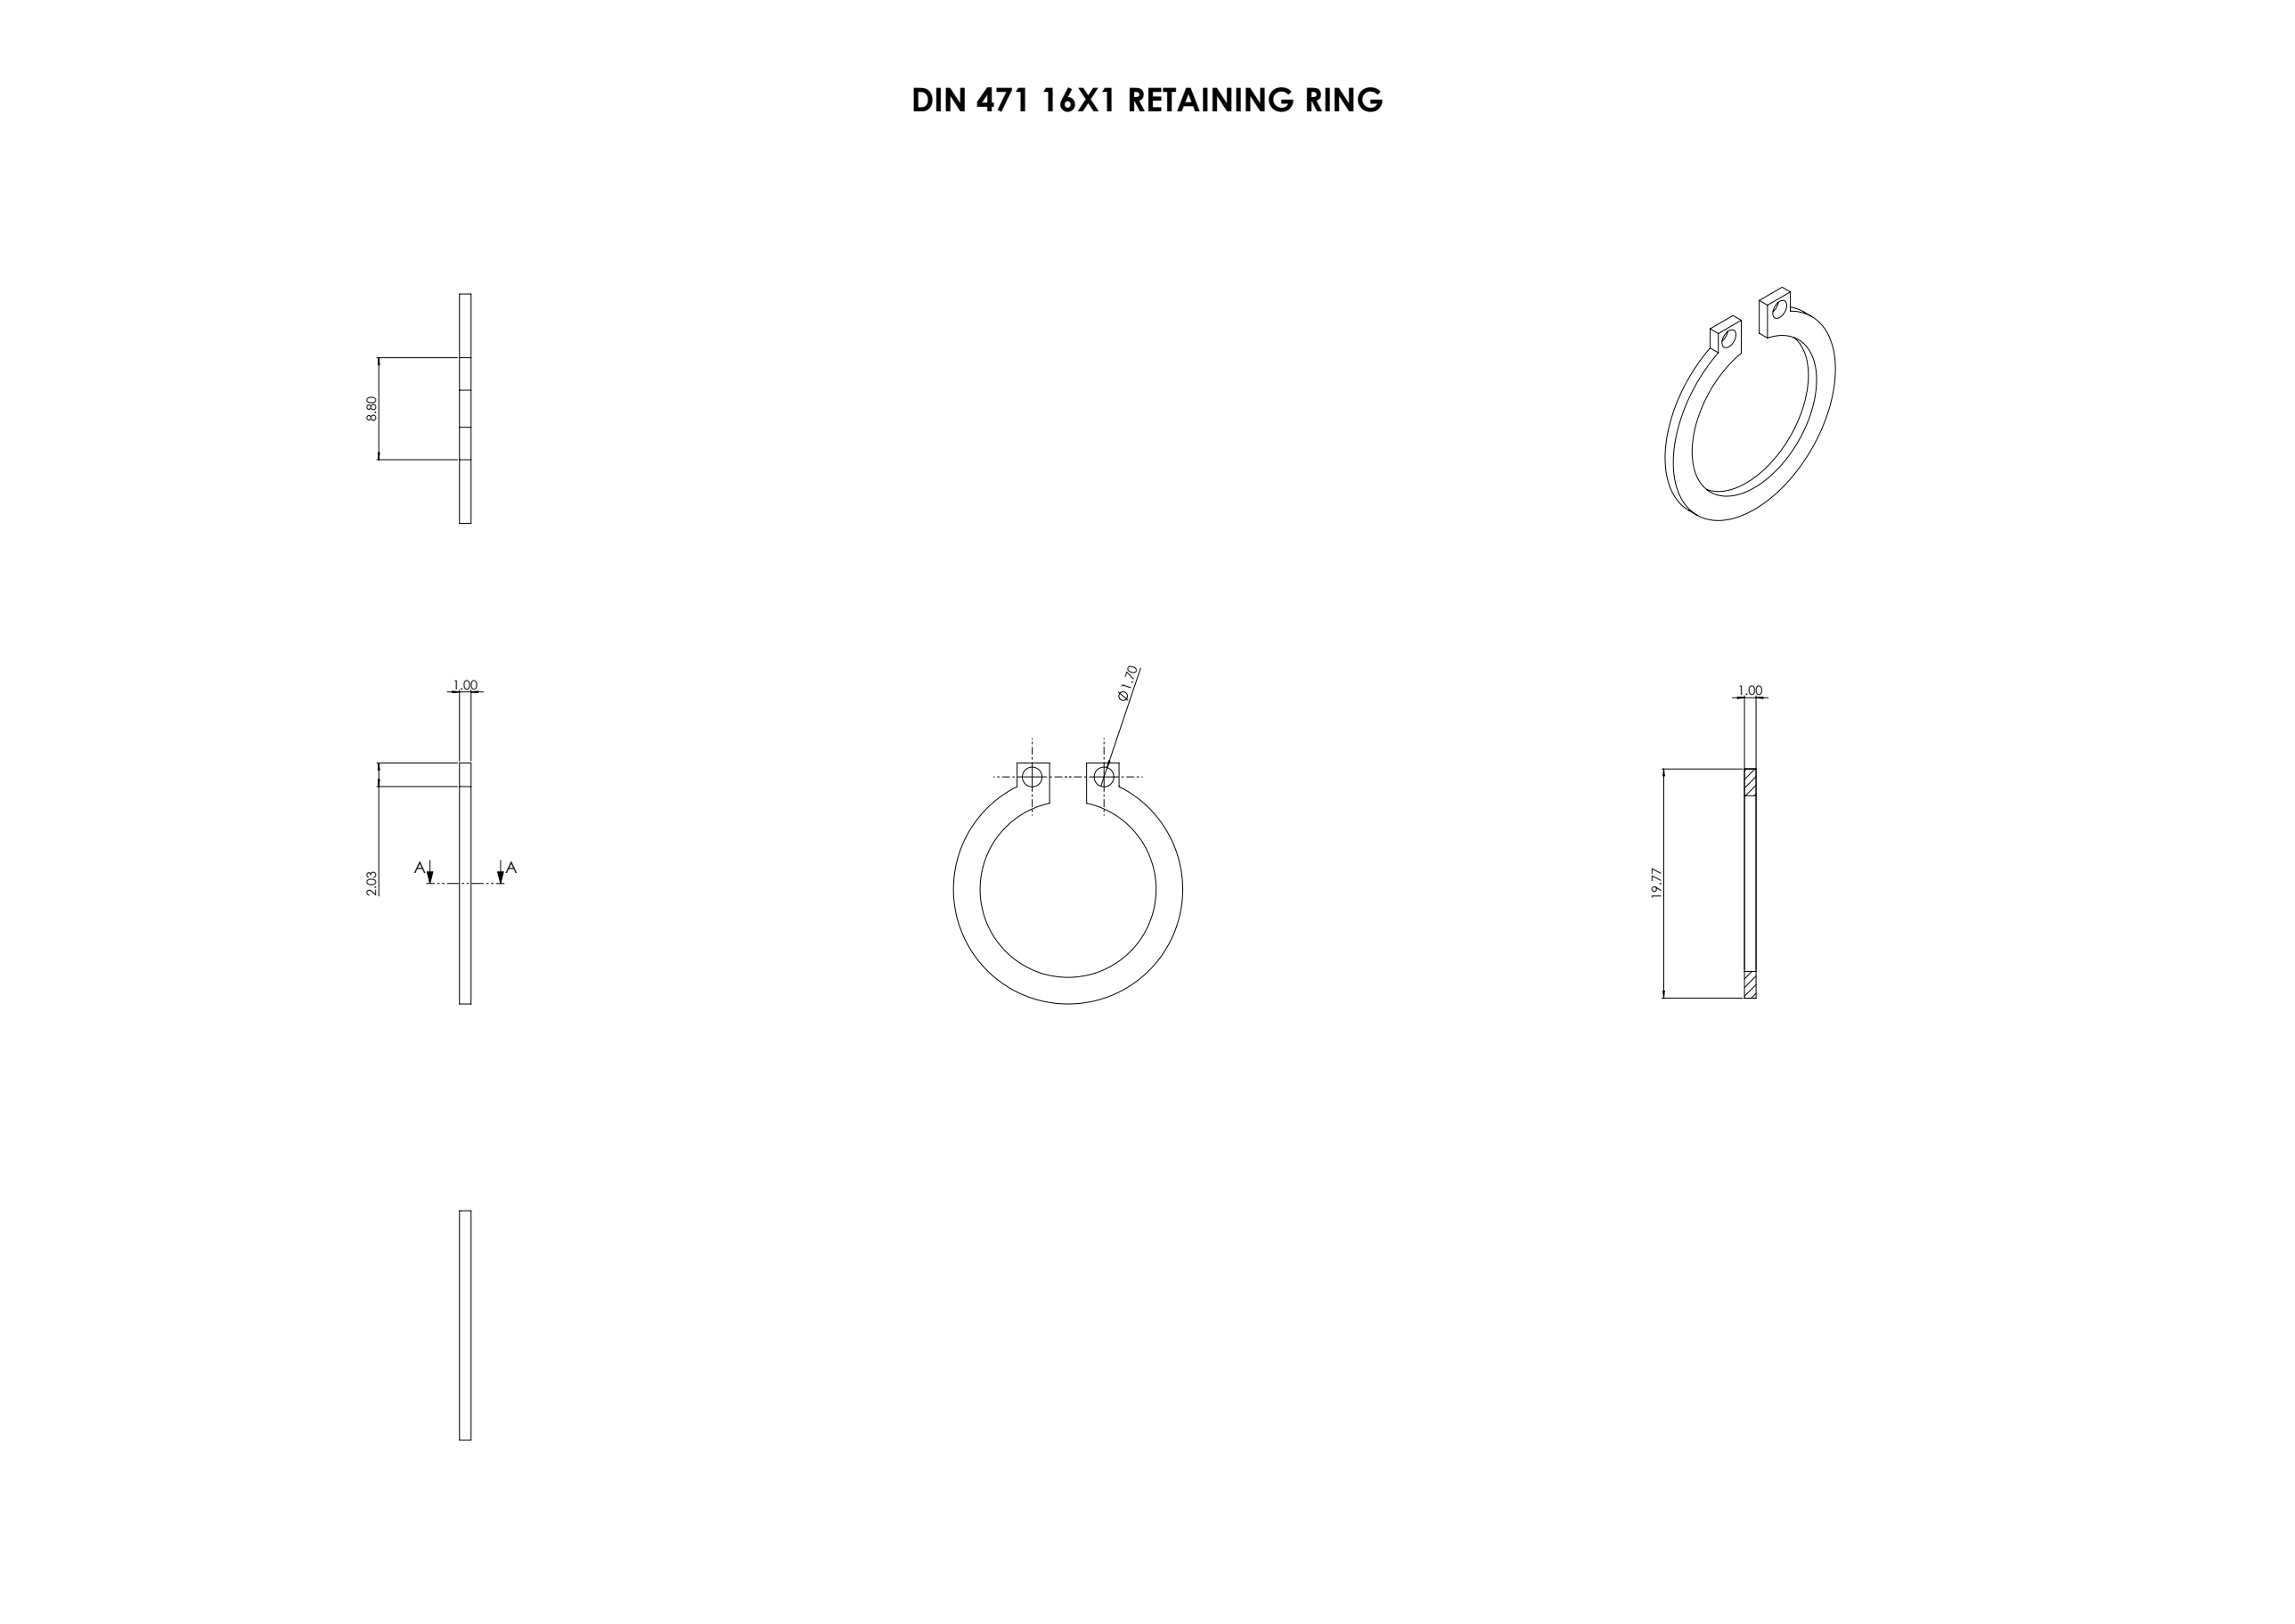
ISO-10303-21;
HEADER;
/* Generated by software containing ST-Developer
 * from STEP Tools, Inc. (www.steptools.com) 
 */

FILE_DESCRIPTION(
/* description */ (''),
/* implementation_level */ '2;1');

FILE_NAME(
/* name */ '09_DIN_471_16x1_Retaining_Ring.step',
/* time_stamp */ '2026-10-24T13:41:11-07:00',
/* author */ (''),
/* organization */ (''),
/* preprocessor_version */ 'ST-DEVELOPER v20.2',
/* originating_system */ 'Autodesk Translation Framework v15.15.0.0',
/* authorisation */ '');

FILE_SCHEMA (('AUTOMOTIVE_DESIGN { 1 0 10303 214 3 1 1 }'));
ENDSEC;

DATA;
#10=MECHANICAL_DESIGN_GEOMETRIC_PRESENTATION_REPRESENTATION('',(#129),#12813);
#109=SHAPE_REPRESENTATION_RELATIONSHIP('SRR','None',#12862,#119);
#119=ADVANCED_BREP_SHAPE_REPRESENTATION('',(#139),#12811);
#129=STYLED_ITEM('',(#12988),#139);
#139=MANIFOLD_SOLID_BREP('Body1',#4392);
#165=FACE_BOUND('',#853,.T.);
#166=FACE_BOUND('',#854,.T.);
#167=FACE_BOUND('',#859,.T.);
#168=FACE_BOUND('',#860,.T.);
#224=PLANE('',#4950);
#225=PLANE('',#4953);
#226=PLANE('',#4954);
#227=PLANE('',#4955);
#228=PLANE('',#4956);
#229=PLANE('',#4960);
#230=PLANE('',#4961);
#231=PLANE('',#4962);
#556=FACE_OUTER_BOUND('',#850,.T.);
#557=FACE_OUTER_BOUND('',#851,.T.);
#558=FACE_OUTER_BOUND('',#852,.T.);
#559=FACE_OUTER_BOUND('',#855,.T.);
#560=FACE_OUTER_BOUND('',#856,.T.);
#561=FACE_OUTER_BOUND('',#857,.T.);
#562=FACE_OUTER_BOUND('',#858,.T.);
#563=FACE_OUTER_BOUND('',#861,.T.);
#564=FACE_OUTER_BOUND('',#862,.T.);
#565=FACE_OUTER_BOUND('',#863,.T.);
#566=FACE_OUTER_BOUND('',#864,.T.);
#567=FACE_OUTER_BOUND('',#865,.T.);
#850=EDGE_LOOP('',(#3873,#3874,#3875,#3876));
#851=EDGE_LOOP('',(#3877,#3878,#3879,#3880));
#852=EDGE_LOOP('',(#3881,#3882,#3883,#3884,#3885,#3886,#3887,#3888));
#853=EDGE_LOOP('',(#3889));
#854=EDGE_LOOP('',(#3890));
#855=EDGE_LOOP('',(#3891,#3892,#3893,#3894));
#856=EDGE_LOOP('',(#3895,#3896,#3897,#3898));
#857=EDGE_LOOP('',(#3899,#3900,#3901,#3902));
#858=EDGE_LOOP('',(#3903,#3904,#3905,#3906,#3907,#3908,#3909,#3910));
#859=EDGE_LOOP('',(#3911));
#860=EDGE_LOOP('',(#3912));
#861=EDGE_LOOP('',(#3913,#3914,#3915,#3916));
#862=EDGE_LOOP('',(#3917,#3918,#3919,#3920));
#863=EDGE_LOOP('',(#3921,#3922,#3923,#3924));
#864=EDGE_LOOP('',(#3925,#3926,#3927,#3928));
#865=EDGE_LOOP('',(#3929,#3930,#3931,#3932));
#1115=CIRCLE('',#4945,0.85);
#1116=CIRCLE('',#4946,0.85);
#1117=CIRCLE('',#4948,0.85);
#1118=CIRCLE('',#4949,0.85);
#1119=CIRCLE('',#4951,9.9);
#1120=CIRCLE('',#4952,7.6);
#1121=CIRCLE('',#4957,7.6);
#1122=CIRCLE('',#4958,9.9);
#1283=LINE('',#12620,#1513);
#1284=LINE('',#12626,#1514);
#1285=LINE('',#12631,#1515);
#1286=LINE('',#12633,#1516);
#1287=LINE('',#12635,#1517);
#1288=LINE('',#12639,#1518);
#1289=LINE('',#12641,#1519);
#1290=LINE('',#12643,#1520);
#1291=LINE('',#12647,#1521);
#1292=LINE('',#12649,#1522);
#1293=LINE('',#12650,#1523);
#1294=LINE('',#12653,#1524);
#1295=LINE('',#12654,#1525);
#1296=LINE('',#12657,#1526);
#1297=LINE('',#12658,#1527);
#1298=LINE('',#12662,#1528);
#1299=LINE('',#12667,#1529);
#1300=LINE('',#12668,#1530);
#1301=LINE('',#12670,#1531);
#1302=LINE('',#12672,#1532);
#1303=LINE('',#12674,#1533);
#1304=LINE('',#12675,#1534);
#1513=VECTOR('',#6046,0.85);
#1514=VECTOR('',#6053,0.85);
#1515=VECTOR('',#6058,10.);
#1516=VECTOR('',#6059,10.);
#1517=VECTOR('',#6060,10.);
#1518=VECTOR('',#6063,10.);
#1519=VECTOR('',#6064,10.);
#1520=VECTOR('',#6065,10.);
#1521=VECTOR('',#6070,10.);
#1522=VECTOR('',#6071,10.);
#1523=VECTOR('',#6072,10.);
#1524=VECTOR('',#6075,10.);
#1525=VECTOR('',#6076,10.);
#1526=VECTOR('',#6079,10.);
#1527=VECTOR('',#6080,10.);
#1528=VECTOR('',#6083,10.);
#1529=VECTOR('',#6088,10.);
#1530=VECTOR('',#6089,10.);
#1531=VECTOR('',#6092,10.);
#1532=VECTOR('',#6095,10.);
#1533=VECTOR('',#6098,10.);
#1534=VECTOR('',#6099,10.);
#2092=VERTEX_POINT('',#12617);
#2093=VERTEX_POINT('',#12619);
#2094=VERTEX_POINT('',#12623);
#2095=VERTEX_POINT('',#12625);
#2096=VERTEX_POINT('',#12629);
#2097=VERTEX_POINT('',#12630);
#2098=VERTEX_POINT('',#12632);
#2099=VERTEX_POINT('',#12634);
#2100=VERTEX_POINT('',#12636);
#2101=VERTEX_POINT('',#12638);
#2102=VERTEX_POINT('',#12640);
#2103=VERTEX_POINT('',#12642);
#2104=VERTEX_POINT('',#12646);
#2105=VERTEX_POINT('',#12648);
#2106=VERTEX_POINT('',#12652);
#2107=VERTEX_POINT('',#12656);
#2108=VERTEX_POINT('',#12660);
#2109=VERTEX_POINT('',#12661);
#2110=VERTEX_POINT('',#12664);
#2111=VERTEX_POINT('',#12666);
#2689=EDGE_CURVE('',#2092,#2092,#1115,.T.);
#2690=EDGE_CURVE('',#2092,#2093,#1283,.T.);
#2691=EDGE_CURVE('',#2093,#2093,#1116,.T.);
#2692=EDGE_CURVE('',#2094,#2094,#1117,.T.);
#2693=EDGE_CURVE('',#2094,#2095,#1284,.T.);
#2694=EDGE_CURVE('',#2095,#2095,#1118,.T.);
#2695=EDGE_CURVE('',#2096,#2097,#1285,.T.);
#2696=EDGE_CURVE('',#2097,#2098,#1286,.T.);
#2697=EDGE_CURVE('',#2098,#2099,#1287,.T.);
#2698=EDGE_CURVE('',#2099,#2100,#1119,.T.);
#2699=EDGE_CURVE('',#2100,#2101,#1288,.T.);
#2700=EDGE_CURVE('',#2101,#2102,#1289,.T.);
#2701=EDGE_CURVE('',#2102,#2103,#1290,.T.);
#2702=EDGE_CURVE('',#2096,#2103,#1120,.T.);
#2703=EDGE_CURVE('',#2104,#2102,#1291,.T.);
#2704=EDGE_CURVE('',#2105,#2104,#1292,.T.);
#2705=EDGE_CURVE('',#2103,#2105,#1293,.T.);
#2706=EDGE_CURVE('',#2104,#2106,#1294,.T.);
#2707=EDGE_CURVE('',#2106,#2101,#1295,.T.);
#2708=EDGE_CURVE('',#2107,#2100,#1296,.T.);
#2709=EDGE_CURVE('',#2106,#2107,#1297,.T.);
#2710=EDGE_CURVE('',#2108,#2109,#1298,.T.);
#2711=EDGE_CURVE('',#2109,#2105,#1121,.T.);
#2712=EDGE_CURVE('',#2110,#2107,#1122,.T.);
#2713=EDGE_CURVE('',#2111,#2110,#1299,.T.);
#2714=EDGE_CURVE('',#2108,#2111,#1300,.T.);
#2715=EDGE_CURVE('',#2099,#2110,#1301,.T.);
#2716=EDGE_CURVE('',#2111,#2098,#1302,.T.);
#2717=EDGE_CURVE('',#2108,#2097,#1303,.T.);
#2718=EDGE_CURVE('',#2109,#2096,#1304,.T.);
#3873=ORIENTED_EDGE('',*,*,#2689,.F.);
#3874=ORIENTED_EDGE('',*,*,#2690,.T.);
#3875=ORIENTED_EDGE('',*,*,#2691,.F.);
#3876=ORIENTED_EDGE('',*,*,#2690,.F.);
#3877=ORIENTED_EDGE('',*,*,#2692,.F.);
#3878=ORIENTED_EDGE('',*,*,#2693,.T.);
#3879=ORIENTED_EDGE('',*,*,#2694,.F.);
#3880=ORIENTED_EDGE('',*,*,#2693,.F.);
#3881=ORIENTED_EDGE('',*,*,#2695,.T.);
#3882=ORIENTED_EDGE('',*,*,#2696,.T.);
#3883=ORIENTED_EDGE('',*,*,#2697,.T.);
#3884=ORIENTED_EDGE('',*,*,#2698,.T.);
#3885=ORIENTED_EDGE('',*,*,#2699,.T.);
#3886=ORIENTED_EDGE('',*,*,#2700,.T.);
#3887=ORIENTED_EDGE('',*,*,#2701,.T.);
#3888=ORIENTED_EDGE('',*,*,#2702,.F.);
#3889=ORIENTED_EDGE('',*,*,#2694,.T.);
#3890=ORIENTED_EDGE('',*,*,#2691,.T.);
#3891=ORIENTED_EDGE('',*,*,#2701,.F.);
#3892=ORIENTED_EDGE('',*,*,#2703,.F.);
#3893=ORIENTED_EDGE('',*,*,#2704,.F.);
#3894=ORIENTED_EDGE('',*,*,#2705,.F.);
#3895=ORIENTED_EDGE('',*,*,#2706,.F.);
#3896=ORIENTED_EDGE('',*,*,#2703,.T.);
#3897=ORIENTED_EDGE('',*,*,#2700,.F.);
#3898=ORIENTED_EDGE('',*,*,#2707,.F.);
#3899=ORIENTED_EDGE('',*,*,#2708,.F.);
#3900=ORIENTED_EDGE('',*,*,#2709,.F.);
#3901=ORIENTED_EDGE('',*,*,#2707,.T.);
#3902=ORIENTED_EDGE('',*,*,#2699,.F.);
#3903=ORIENTED_EDGE('',*,*,#2710,.T.);
#3904=ORIENTED_EDGE('',*,*,#2711,.T.);
#3905=ORIENTED_EDGE('',*,*,#2704,.T.);
#3906=ORIENTED_EDGE('',*,*,#2706,.T.);
#3907=ORIENTED_EDGE('',*,*,#2709,.T.);
#3908=ORIENTED_EDGE('',*,*,#2712,.F.);
#3909=ORIENTED_EDGE('',*,*,#2713,.F.);
#3910=ORIENTED_EDGE('',*,*,#2714,.F.);
#3911=ORIENTED_EDGE('',*,*,#2689,.T.);
#3912=ORIENTED_EDGE('',*,*,#2692,.T.);
#3913=ORIENTED_EDGE('',*,*,#2708,.T.);
#3914=ORIENTED_EDGE('',*,*,#2698,.F.);
#3915=ORIENTED_EDGE('',*,*,#2715,.T.);
#3916=ORIENTED_EDGE('',*,*,#2712,.T.);
#3917=ORIENTED_EDGE('',*,*,#2715,.F.);
#3918=ORIENTED_EDGE('',*,*,#2697,.F.);
#3919=ORIENTED_EDGE('',*,*,#2716,.F.);
#3920=ORIENTED_EDGE('',*,*,#2713,.T.);
#3921=ORIENTED_EDGE('',*,*,#2710,.F.);
#3922=ORIENTED_EDGE('',*,*,#2717,.T.);
#3923=ORIENTED_EDGE('',*,*,#2695,.F.);
#3924=ORIENTED_EDGE('',*,*,#2718,.F.);
#3925=ORIENTED_EDGE('',*,*,#2714,.T.);
#3926=ORIENTED_EDGE('',*,*,#2716,.T.);
#3927=ORIENTED_EDGE('',*,*,#2696,.F.);
#3928=ORIENTED_EDGE('',*,*,#2717,.F.);
#3929=ORIENTED_EDGE('',*,*,#2718,.T.);
#3930=ORIENTED_EDGE('',*,*,#2702,.T.);
#3931=ORIENTED_EDGE('',*,*,#2705,.T.);
#3932=ORIENTED_EDGE('',*,*,#2711,.F.);
#4110=CYLINDRICAL_SURFACE('',#4944,0.85);
#4111=CYLINDRICAL_SURFACE('',#4947,0.85);
#4112=CYLINDRICAL_SURFACE('',#4959,9.9);
#4113=CYLINDRICAL_SURFACE('',#4963,7.6);
#4346=ADVANCED_FACE('',(#556),#4110,.F.);
#4347=ADVANCED_FACE('',(#557),#4111,.F.);
#4348=ADVANCED_FACE('',(#558,#165,#166),#224,.T.);
#4349=ADVANCED_FACE('',(#559),#225,.T.);
#4350=ADVANCED_FACE('',(#560),#226,.T.);
#4351=ADVANCED_FACE('',(#561),#227,.T.);
#4352=ADVANCED_FACE('',(#562,#167,#168),#228,.T.);
#4353=ADVANCED_FACE('',(#563),#4112,.T.);
#4354=ADVANCED_FACE('',(#564),#229,.T.);
#4355=ADVANCED_FACE('',(#565),#230,.T.);
#4356=ADVANCED_FACE('',(#566),#231,.T.);
#4357=ADVANCED_FACE('',(#567),#4113,.F.);
#4392=CLOSED_SHELL('',(#4346,#4347,#4348,#4349,#4350,#4351,#4352,#4353,
#4354,#4355,#4356,#4357));
#4943=AXIS2_PLACEMENT_3D('',#12615,#6040,#6041);
#4944=AXIS2_PLACEMENT_3D('',#12616,#6042,#6043);
#4945=AXIS2_PLACEMENT_3D('',#12618,#6044,#6045);
#4946=AXIS2_PLACEMENT_3D('',#12621,#6047,#6048);
#4947=AXIS2_PLACEMENT_3D('',#12622,#6049,#6050);
#4948=AXIS2_PLACEMENT_3D('',#12624,#6051,#6052);
#4949=AXIS2_PLACEMENT_3D('',#12627,#6054,#6055);
#4950=AXIS2_PLACEMENT_3D('',#12628,#6056,#6057);
#4951=AXIS2_PLACEMENT_3D('',#12637,#6061,#6062);
#4952=AXIS2_PLACEMENT_3D('',#12644,#6066,#6067);
#4953=AXIS2_PLACEMENT_3D('',#12645,#6068,#6069);
#4954=AXIS2_PLACEMENT_3D('',#12651,#6073,#6074);
#4955=AXIS2_PLACEMENT_3D('',#12655,#6077,#6078);
#4956=AXIS2_PLACEMENT_3D('',#12659,#6081,#6082);
#4957=AXIS2_PLACEMENT_3D('',#12663,#6084,#6085);
#4958=AXIS2_PLACEMENT_3D('',#12665,#6086,#6087);
#4959=AXIS2_PLACEMENT_3D('',#12669,#6090,#6091);
#4960=AXIS2_PLACEMENT_3D('',#12671,#6093,#6094);
#4961=AXIS2_PLACEMENT_3D('',#12673,#6096,#6097);
#4962=AXIS2_PLACEMENT_3D('',#12676,#6100,#6101);
#4963=AXIS2_PLACEMENT_3D('',#12677,#6102,#6103);
#6040=DIRECTION('axis',(0.,0.,1.));
#6041=DIRECTION('refdir',(1.,0.,0.));
#6042=DIRECTION('center_axis',(1.,0.,0.));
#6043=DIRECTION('ref_axis',(0.,0.,-1.));
#6044=DIRECTION('center_axis',(1.,0.,0.));
#6045=DIRECTION('ref_axis',(0.,0.,-1.));
#6046=DIRECTION('',(1.,0.,0.));
#6047=DIRECTION('center_axis',(-1.,0.,0.));
#6048=DIRECTION('ref_axis',(0.,0.,-1.));
#6049=DIRECTION('center_axis',(1.,0.,0.));
#6050=DIRECTION('ref_axis',(0.,0.,-1.));
#6051=DIRECTION('center_axis',(1.,0.,0.));
#6052=DIRECTION('ref_axis',(0.,0.,-1.));
#6053=DIRECTION('',(1.,0.,0.));
#6054=DIRECTION('center_axis',(-1.,0.,0.));
#6055=DIRECTION('ref_axis',(0.,0.,-1.));
#6056=DIRECTION('center_axis',(1.,0.,0.));
#6057=DIRECTION('ref_axis',(0.,0.,-1.));
#6058=DIRECTION('',(0.,1.,0.));
#6059=DIRECTION('',(0.,0.,1.));
#6060=DIRECTION('',(0.,-1.,0.));
#6061=DIRECTION('center_axis',(1.,0.,0.));
#6062=DIRECTION('ref_axis',(0.,0.,-1.));
#6063=DIRECTION('',(0.,1.,0.));
#6064=DIRECTION('',(0.,0.,1.));
#6065=DIRECTION('',(0.,-1.,0.));
#6066=DIRECTION('center_axis',(1.,0.,0.));
#6067=DIRECTION('ref_axis',(0.,0.,-1.));
#6068=DIRECTION('center_axis',(0.,0.,1.));
#6069=DIRECTION('ref_axis',(0.,-1.,0.));
#6070=DIRECTION('',(1.,0.,0.));
#6071=DIRECTION('',(0.,1.,0.));
#6072=DIRECTION('',(-1.,0.,0.));
#6073=DIRECTION('center_axis',(0.,1.,0.));
#6074=DIRECTION('ref_axis',(0.,0.,1.));
#6075=DIRECTION('',(0.,0.,-1.));
#6076=DIRECTION('',(1.,0.,0.));
#6077=DIRECTION('center_axis',(0.,0.,-1.));
#6078=DIRECTION('ref_axis',(0.,1.,0.));
#6079=DIRECTION('',(1.,0.,0.));
#6080=DIRECTION('',(0.,-1.,0.));
#6081=DIRECTION('center_axis',(-1.,0.,0.));
#6082=DIRECTION('ref_axis',(0.,0.,1.));
#6083=DIRECTION('',(0.,-1.,0.));
#6084=DIRECTION('center_axis',(1.,0.,0.));
#6085=DIRECTION('ref_axis',(0.,0.,-1.));
#6086=DIRECTION('center_axis',(1.,0.,0.));
#6087=DIRECTION('ref_axis',(0.,0.,-1.));
#6088=DIRECTION('',(0.,-1.,0.));
#6089=DIRECTION('',(0.,0.,1.));
#6090=DIRECTION('center_axis',(1.,0.,0.));
#6091=DIRECTION('ref_axis',(0.,-1.,-1.22464679914735E-16));
#6092=DIRECTION('',(-1.,0.,0.));
#6093=DIRECTION('center_axis',(0.,0.,1.));
#6094=DIRECTION('ref_axis',(0.,-1.,0.));
#6095=DIRECTION('',(1.,0.,0.));
#6096=DIRECTION('center_axis',(0.,0.,-1.));
#6097=DIRECTION('ref_axis',(0.,1.,0.));
#6098=DIRECTION('',(1.,0.,0.));
#6099=DIRECTION('',(1.,0.,0.));
#6100=DIRECTION('center_axis',(0.,1.,0.));
#6101=DIRECTION('ref_axis',(0.,0.,1.));
#6102=DIRECTION('center_axis',(1.,0.,0.));
#6103=DIRECTION('ref_axis',(0.,-1.,1.22464679914735E-16));
#12615=CARTESIAN_POINT('',(0.,0.,0.));
#12616=CARTESIAN_POINT('Origin',(0.,9.7,3.1));
#12617=CARTESIAN_POINT('',(0.,9.7,3.95));
#12618=CARTESIAN_POINT('Origin',(0.,9.7,3.1));
#12619=CARTESIAN_POINT('',(1.,9.7,3.95));
#12620=CARTESIAN_POINT('',(0.,9.7,3.95));
#12621=CARTESIAN_POINT('Origin',(1.,9.7,3.1));
#12622=CARTESIAN_POINT('Origin',(0.,9.7,-3.1));
#12623=CARTESIAN_POINT('',(0.,9.7,-2.25));
#12624=CARTESIAN_POINT('Origin',(0.,9.7,-3.1));
#12625=CARTESIAN_POINT('',(1.,9.7,-2.25));
#12626=CARTESIAN_POINT('',(0.,9.7,-2.25));
#12627=CARTESIAN_POINT('Origin',(1.,9.7,-3.1));
#12628=CARTESIAN_POINT('Origin',(1.,7.6,0.));
#12629=CARTESIAN_POINT('',(1.,7.42967024840268,1.6));
#12630=CARTESIAN_POINT('',(1.,10.9,1.6));
#12631=CARTESIAN_POINT('',(1.,8.3,1.6));
#12632=CARTESIAN_POINT('',(1.,10.9,4.4));
#12633=CARTESIAN_POINT('',(1.,10.9,1.6));
#12634=CARTESIAN_POINT('',(1.,8.8684835231284,4.4));
#12635=CARTESIAN_POINT('',(1.,10.9,4.4));
#12636=CARTESIAN_POINT('',(1.,8.8684835231284,-4.4));
#12637=CARTESIAN_POINT('Origin',(1.,0.,0.));
#12638=CARTESIAN_POINT('',(1.,10.9,-4.4));
#12639=CARTESIAN_POINT('',(1.,10.9,-4.4));
#12640=CARTESIAN_POINT('',(1.,10.9,-1.6));
#12641=CARTESIAN_POINT('',(1.,10.9,-1.6));
#12642=CARTESIAN_POINT('',(1.,7.42967024840268,-1.6));
#12643=CARTESIAN_POINT('',(1.,7.3,-1.6));
#12644=CARTESIAN_POINT('Origin',(1.,0.,0.));
#12645=CARTESIAN_POINT('Origin',(0.,10.9,-1.6));
#12646=CARTESIAN_POINT('',(0.,10.9,-1.6));
#12647=CARTESIAN_POINT('',(0.,10.9,-1.6));
#12648=CARTESIAN_POINT('',(0.,7.42967024840268,-1.6));
#12649=CARTESIAN_POINT('',(0.,8.45,-1.6));
#12650=CARTESIAN_POINT('',(0.5,7.42967024840268,-1.6));
#12651=CARTESIAN_POINT('Origin',(0.,10.9,-4.4));
#12652=CARTESIAN_POINT('',(0.,10.9,-4.4));
#12653=CARTESIAN_POINT('',(0.,10.9,-1.6));
#12654=CARTESIAN_POINT('',(0.,10.9,-4.4));
#12655=CARTESIAN_POINT('Origin',(0.,8.3,-4.4));
#12656=CARTESIAN_POINT('',(0.,8.8684835231284,-4.4));
#12657=CARTESIAN_POINT('',(0.5,8.8684835231284,-4.4));
#12658=CARTESIAN_POINT('',(0.,10.9,-4.4));
#12659=CARTESIAN_POINT('Origin',(0.,9.9,0.));
#12660=CARTESIAN_POINT('',(0.,10.9,1.6));
#12661=CARTESIAN_POINT('',(0.,7.42967024840268,1.6));
#12662=CARTESIAN_POINT('',(0.,10.7,1.6));
#12663=CARTESIAN_POINT('Origin',(0.,0.,0.));
#12664=CARTESIAN_POINT('',(0.,8.8684835231284,4.4));
#12665=CARTESIAN_POINT('Origin',(0.,0.,0.));
#12666=CARTESIAN_POINT('',(0.,10.9,4.4));
#12667=CARTESIAN_POINT('',(0.,10.9,4.4));
#12668=CARTESIAN_POINT('',(0.,10.9,1.6));
#12669=CARTESIAN_POINT('Origin',(0.5,0.,0.));
#12670=CARTESIAN_POINT('',(0.5,8.8684835231284,4.4));
#12671=CARTESIAN_POINT('Origin',(0.,10.9,4.4));
#12672=CARTESIAN_POINT('',(0.,10.9,4.4));
#12673=CARTESIAN_POINT('Origin',(0.,8.3,1.6));
#12674=CARTESIAN_POINT('',(0.,10.9,1.6));
#12675=CARTESIAN_POINT('',(0.5,7.42967024840268,1.6));
#12676=CARTESIAN_POINT('Origin',(0.,10.9,1.6));
#12677=CARTESIAN_POINT('Origin',(0.5,0.,0.));
#12799=UNCERTAINTY_MEASURE_WITH_UNIT(LENGTH_MEASURE(0.01),#12814,
'DISTANCE_ACCURACY_VALUE',
'Maximum model space distance between geometric entities at asserted c
onnectivities');
#12801=UNCERTAINTY_MEASURE_WITH_UNIT(LENGTH_MEASURE(0.01),#12814,
'DISTANCE_ACCURACY_VALUE',
'Maximum model space distance between geometric entities at asserted c
onnectivities');
#12811=(
GEOMETRIC_REPRESENTATION_CONTEXT(3)
GLOBAL_UNCERTAINTY_ASSIGNED_CONTEXT((#12799))
GLOBAL_UNIT_ASSIGNED_CONTEXT((#12814,#12816,#12817))
REPRESENTATION_CONTEXT('','3D')
);
#12813=(
GEOMETRIC_REPRESENTATION_CONTEXT(3)
GLOBAL_UNCERTAINTY_ASSIGNED_CONTEXT((#12801))
GLOBAL_UNIT_ASSIGNED_CONTEXT((#12814,#12816,#12817))
REPRESENTATION_CONTEXT('','3D')
);
#12814=(
LENGTH_UNIT()
NAMED_UNIT(*)
SI_UNIT(.MILLI.,.METRE.)
);
#12816=(
NAMED_UNIT(*)
PLANE_ANGLE_UNIT()
SI_UNIT($,.RADIAN.)
);
#12817=(
NAMED_UNIT(*)
SI_UNIT($,.STERADIAN.)
SOLID_ANGLE_UNIT()
);
#12827=SHAPE_DEFINITION_REPRESENTATION(#12838,#12862);
#12838=PRODUCT_DEFINITION_SHAPE('',$,#12874);
#12862=SHAPE_REPRESENTATION('',(#4943),#12811);
#12864=PRODUCT_DEFINITION_CONTEXT('part definition',#12899,'design');
#12874=PRODUCT_DEFINITION('2026-10-11-12-17-36-454',
'09_DIN_471_16x1_Retaining_Ring',#12885,#12864);
#12885=PRODUCT_DEFINITION_FORMATION('',$,#12910);
#12899=APPLICATION_CONTEXT(
'Core Data for Automotive Mechanical Design Process');
#12900=PRODUCT_CONTEXT('part definition',#12899,'mechanical');
#12910=PRODUCT('2026-10-11-12-17-36-454',
'09_DIN_471_16x1_Retaining_Ring',$,(#12900));
#12982=COLOUR_RGB('Off White',0.89,0.88,0.83);
#12983=FILL_AREA_STYLE_COLOUR('',#12982);
#12984=FILL_AREA_STYLE('',(#12983));
#12985=SURFACE_STYLE_FILL_AREA(#12984);
#12986=SURFACE_SIDE_STYLE('',(#12985));
#12987=SURFACE_STYLE_USAGE(.BOTH.,#12986);
#12988=PRESENTATION_STYLE_ASSIGNMENT((#12987));
ENDSEC;
END-ISO-10303-21;
